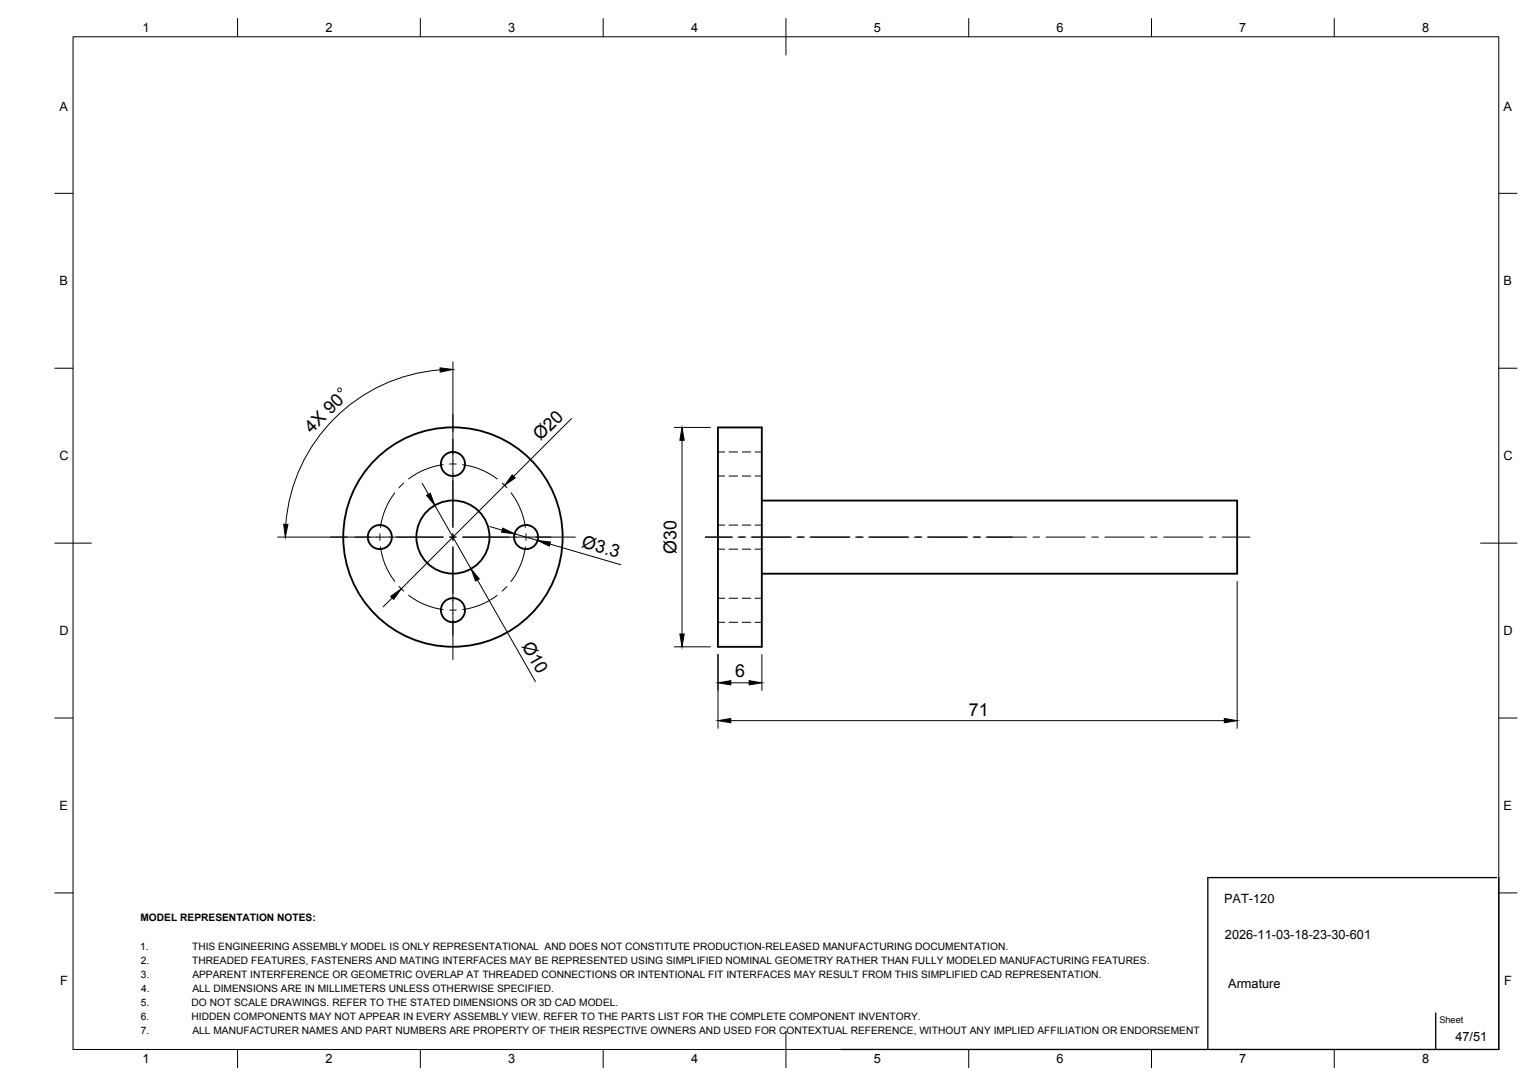
ISO-10303-21;
HEADER;
/* Generated by software containing ST-Developer
 * from STEP Tools, Inc. (www.steptools.com) 
 */

FILE_DESCRIPTION(
/* description */ ('Vibration shaker table dummy'),
/* implementation_level */ '2;1');

FILE_NAME(
/* name */ 'Armature.step',
/* time_stamp */ '2026-10-27T10:55:14-07:00',
/* author */ (''),
/* organization */ (''),
/* preprocessor_version */ 'ST-DEVELOPER v20.2',
/* originating_system */ 'Autodesk Translation Framework v15.17.0.0',
/* authorisation */ '');

FILE_SCHEMA (('AUTOMOTIVE_DESIGN { 1 0 10303 214 3 1 1 }'));
ENDSEC;

DATA;
#10=MECHANICAL_DESIGN_GEOMETRIC_PRESENTATION_REPRESENTATION('',(#728),#22394);
#636=SHAPE_REPRESENTATION_RELATIONSHIP('SRR','None',#22683,#682);
#682=ADVANCED_BREP_SHAPE_REPRESENTATION('',(#772),#22389);
#728=STYLED_ITEM('',(#22947),#772);
#772=MANIFOLD_SOLID_BREP('Body1',#9248);
#1039=FACE_BOUND('',#2555,.T.);
#1040=FACE_BOUND('',#2556,.T.);
#1041=FACE_BOUND('',#2557,.T.);
#1042=FACE_BOUND('',#2558,.T.);
#1043=FACE_BOUND('',#2559,.T.);
#1044=FACE_BOUND('',#2563,.T.);
#1045=FACE_BOUND('',#2564,.T.);
#1046=FACE_BOUND('',#2565,.T.);
#1047=FACE_BOUND('',#2566,.T.);
#1310=PLANE('',#10726);
#1311=PLANE('',#10733);
#1312=PLANE('',#10734);
#1788=FACE_OUTER_BOUND('',#2550,.T.);
#1789=FACE_OUTER_BOUND('',#2551,.T.);
#1790=FACE_OUTER_BOUND('',#2552,.T.);
#1791=FACE_OUTER_BOUND('',#2553,.T.);
#1792=FACE_OUTER_BOUND('',#2554,.T.);
#1793=FACE_OUTER_BOUND('',#2560,.T.);
#1794=FACE_OUTER_BOUND('',#2561,.T.);
#1795=FACE_OUTER_BOUND('',#2562,.T.);
#1796=FACE_OUTER_BOUND('',#2567,.T.);
#2550=EDGE_LOOP('',(#8310,#8311,#8312,#8313));
#2551=EDGE_LOOP('',(#8314,#8315,#8316,#8317));
#2552=EDGE_LOOP('',(#8318,#8319,#8320,#8321));
#2553=EDGE_LOOP('',(#8322,#8323,#8324,#8325));
#2554=EDGE_LOOP('',(#8326));
#2555=EDGE_LOOP('',(#8327));
#2556=EDGE_LOOP('',(#8328));
#2557=EDGE_LOOP('',(#8329));
#2558=EDGE_LOOP('',(#8330));
#2559=EDGE_LOOP('',(#8331));
#2560=EDGE_LOOP('',(#8332,#8333,#8334,#8335));
#2561=EDGE_LOOP('',(#8336,#8337,#8338,#8339));
#2562=EDGE_LOOP('',(#8340));
#2563=EDGE_LOOP('',(#8341));
#2564=EDGE_LOOP('',(#8342));
#2565=EDGE_LOOP('',(#8343));
#2566=EDGE_LOOP('',(#8344));
#2567=EDGE_LOOP('',(#8345));
#3185=LINE('',#21941,#3804);
#3186=LINE('',#21947,#3805);
#3187=LINE('',#21953,#3806);
#3188=LINE('',#21959,#3807);
#3189=LINE('',#21969,#3808);
#3190=LINE('',#21972,#3809);
#3804=VECTOR('',#13425,0.165);
#3805=VECTOR('',#13432,0.165);
#3806=VECTOR('',#13439,0.165);
#3807=VECTOR('',#13446,0.165);
#3808=VECTOR('',#13459,1.5);
#3809=VECTOR('',#13462,0.5);
#4325=CIRCLE('',#10715,0.165);
#4326=CIRCLE('',#10716,0.165);
#4327=CIRCLE('',#10718,0.165);
#4328=CIRCLE('',#10719,0.165);
#4329=CIRCLE('',#10721,0.165);
#4330=CIRCLE('',#10722,0.165);
#4331=CIRCLE('',#10724,0.165);
#4332=CIRCLE('',#10725,0.165);
#4333=CIRCLE('',#10727,1.5);
#4334=CIRCLE('',#10728,0.5);
#4335=CIRCLE('',#10730,1.5);
#4336=CIRCLE('',#10732,0.5);
#5052=VERTEX_POINT('',#21938);
#5053=VERTEX_POINT('',#21940);
#5054=VERTEX_POINT('',#21944);
#5055=VERTEX_POINT('',#21946);
#5056=VERTEX_POINT('',#21950);
#5057=VERTEX_POINT('',#21952);
#5058=VERTEX_POINT('',#21956);
#5059=VERTEX_POINT('',#21958);
#5060=VERTEX_POINT('',#21962);
#5061=VERTEX_POINT('',#21964);
#5062=VERTEX_POINT('',#21967);
#5063=VERTEX_POINT('',#21971);
#6148=EDGE_CURVE('',#5052,#5052,#4325,.T.);
#6149=EDGE_CURVE('',#5052,#5053,#3185,.T.);
#6150=EDGE_CURVE('',#5053,#5053,#4326,.T.);
#6151=EDGE_CURVE('',#5054,#5054,#4327,.T.);
#6152=EDGE_CURVE('',#5054,#5055,#3186,.T.);
#6153=EDGE_CURVE('',#5055,#5055,#4328,.T.);
#6154=EDGE_CURVE('',#5056,#5056,#4329,.T.);
#6155=EDGE_CURVE('',#5056,#5057,#3187,.T.);
#6156=EDGE_CURVE('',#5057,#5057,#4330,.T.);
#6157=EDGE_CURVE('',#5058,#5058,#4331,.T.);
#6158=EDGE_CURVE('',#5058,#5059,#3188,.T.);
#6159=EDGE_CURVE('',#5059,#5059,#4332,.T.);
#6160=EDGE_CURVE('',#5060,#5060,#4333,.T.);
#6161=EDGE_CURVE('',#5061,#5061,#4334,.T.);
#6162=EDGE_CURVE('',#5062,#5062,#4335,.T.);
#6163=EDGE_CURVE('',#5062,#5060,#3189,.T.);
#6164=EDGE_CURVE('',#5061,#5063,#3190,.T.);
#6165=EDGE_CURVE('',#5063,#5063,#4336,.T.);
#8310=ORIENTED_EDGE('',*,*,#6148,.F.);
#8311=ORIENTED_EDGE('',*,*,#6149,.T.);
#8312=ORIENTED_EDGE('',*,*,#6150,.F.);
#8313=ORIENTED_EDGE('',*,*,#6149,.F.);
#8314=ORIENTED_EDGE('',*,*,#6151,.F.);
#8315=ORIENTED_EDGE('',*,*,#6152,.T.);
#8316=ORIENTED_EDGE('',*,*,#6153,.F.);
#8317=ORIENTED_EDGE('',*,*,#6152,.F.);
#8318=ORIENTED_EDGE('',*,*,#6154,.F.);
#8319=ORIENTED_EDGE('',*,*,#6155,.T.);
#8320=ORIENTED_EDGE('',*,*,#6156,.F.);
#8321=ORIENTED_EDGE('',*,*,#6155,.F.);
#8322=ORIENTED_EDGE('',*,*,#6157,.F.);
#8323=ORIENTED_EDGE('',*,*,#6158,.T.);
#8324=ORIENTED_EDGE('',*,*,#6159,.F.);
#8325=ORIENTED_EDGE('',*,*,#6158,.F.);
#8326=ORIENTED_EDGE('',*,*,#6160,.F.);
#8327=ORIENTED_EDGE('',*,*,#6161,.F.);
#8328=ORIENTED_EDGE('',*,*,#6157,.T.);
#8329=ORIENTED_EDGE('',*,*,#6154,.T.);
#8330=ORIENTED_EDGE('',*,*,#6151,.T.);
#8331=ORIENTED_EDGE('',*,*,#6148,.T.);
#8332=ORIENTED_EDGE('',*,*,#6162,.F.);
#8333=ORIENTED_EDGE('',*,*,#6163,.T.);
#8334=ORIENTED_EDGE('',*,*,#6160,.T.);
#8335=ORIENTED_EDGE('',*,*,#6163,.F.);
#8336=ORIENTED_EDGE('',*,*,#6161,.T.);
#8337=ORIENTED_EDGE('',*,*,#6164,.T.);
#8338=ORIENTED_EDGE('',*,*,#6165,.T.);
#8339=ORIENTED_EDGE('',*,*,#6164,.F.);
#8340=ORIENTED_EDGE('',*,*,#6162,.T.);
#8341=ORIENTED_EDGE('',*,*,#6150,.T.);
#8342=ORIENTED_EDGE('',*,*,#6153,.T.);
#8343=ORIENTED_EDGE('',*,*,#6156,.T.);
#8344=ORIENTED_EDGE('',*,*,#6159,.T.);
#8345=ORIENTED_EDGE('',*,*,#6165,.F.);
#8690=CYLINDRICAL_SURFACE('',#10714,0.165);
#8691=CYLINDRICAL_SURFACE('',#10717,0.165);
#8692=CYLINDRICAL_SURFACE('',#10720,0.165);
#8693=CYLINDRICAL_SURFACE('',#10723,0.165);
#8694=CYLINDRICAL_SURFACE('',#10729,1.5);
#8695=CYLINDRICAL_SURFACE('',#10731,0.5);
#9153=ADVANCED_FACE('',(#1788),#8690,.F.);
#9154=ADVANCED_FACE('',(#1789),#8691,.F.);
#9155=ADVANCED_FACE('',(#1790),#8692,.F.);
#9156=ADVANCED_FACE('',(#1791),#8693,.F.);
#9157=ADVANCED_FACE('',(#1792,#1039,#1040,#1041,#1042,#1043),#1310,.F.);
#9158=ADVANCED_FACE('',(#1793),#8694,.T.);
#9159=ADVANCED_FACE('',(#1794),#8695,.T.);
#9160=ADVANCED_FACE('',(#1795,#1044,#1045,#1046,#1047),#1311,.T.);
#9161=ADVANCED_FACE('',(#1796),#1312,.F.);
#9248=CLOSED_SHELL('',(#9153,#9154,#9155,#9156,#9157,#9158,#9159,#9160,
#9161));
#10713=AXIS2_PLACEMENT_3D('',#21936,#13419,#13420);
#10714=AXIS2_PLACEMENT_3D('',#21937,#13421,#13422);
#10715=AXIS2_PLACEMENT_3D('',#21939,#13423,#13424);
#10716=AXIS2_PLACEMENT_3D('',#21942,#13426,#13427);
#10717=AXIS2_PLACEMENT_3D('',#21943,#13428,#13429);
#10718=AXIS2_PLACEMENT_3D('',#21945,#13430,#13431);
#10719=AXIS2_PLACEMENT_3D('',#21948,#13433,#13434);
#10720=AXIS2_PLACEMENT_3D('',#21949,#13435,#13436);
#10721=AXIS2_PLACEMENT_3D('',#21951,#13437,#13438);
#10722=AXIS2_PLACEMENT_3D('',#21954,#13440,#13441);
#10723=AXIS2_PLACEMENT_3D('',#21955,#13442,#13443);
#10724=AXIS2_PLACEMENT_3D('',#21957,#13444,#13445);
#10725=AXIS2_PLACEMENT_3D('',#21960,#13447,#13448);
#10726=AXIS2_PLACEMENT_3D('',#21961,#13449,#13450);
#10727=AXIS2_PLACEMENT_3D('',#21963,#13451,#13452);
#10728=AXIS2_PLACEMENT_3D('',#21965,#13453,#13454);
#10729=AXIS2_PLACEMENT_3D('',#21966,#13455,#13456);
#10730=AXIS2_PLACEMENT_3D('',#21968,#13457,#13458);
#10731=AXIS2_PLACEMENT_3D('',#21970,#13460,#13461);
#10732=AXIS2_PLACEMENT_3D('',#21973,#13463,#13464);
#10733=AXIS2_PLACEMENT_3D('',#21974,#13465,#13466);
#10734=AXIS2_PLACEMENT_3D('',#21975,#13467,#13468);
#13419=DIRECTION('axis',(0.,0.,1.));
#13420=DIRECTION('refdir',(1.,0.,0.));
#13421=DIRECTION('center_axis',(0.,0.,1.));
#13422=DIRECTION('ref_axis',(1.,0.,0.));
#13423=DIRECTION('center_axis',(0.,0.,1.));
#13424=DIRECTION('ref_axis',(1.,0.,0.));
#13425=DIRECTION('',(0.,0.,1.));
#13426=DIRECTION('center_axis',(0.,0.,-1.));
#13427=DIRECTION('ref_axis',(1.,0.,0.));
#13428=DIRECTION('center_axis',(0.,0.,1.));
#13429=DIRECTION('ref_axis',(1.,0.,0.));
#13430=DIRECTION('center_axis',(0.,0.,1.));
#13431=DIRECTION('ref_axis',(1.,0.,0.));
#13432=DIRECTION('',(0.,0.,1.));
#13433=DIRECTION('center_axis',(0.,0.,-1.));
#13434=DIRECTION('ref_axis',(1.,0.,0.));
#13435=DIRECTION('center_axis',(0.,0.,1.));
#13436=DIRECTION('ref_axis',(1.,0.,0.));
#13437=DIRECTION('center_axis',(0.,0.,1.));
#13438=DIRECTION('ref_axis',(1.,0.,0.));
#13439=DIRECTION('',(0.,0.,1.));
#13440=DIRECTION('center_axis',(0.,0.,-1.));
#13441=DIRECTION('ref_axis',(1.,0.,0.));
#13442=DIRECTION('center_axis',(0.,0.,1.));
#13443=DIRECTION('ref_axis',(1.,0.,0.));
#13444=DIRECTION('center_axis',(0.,0.,1.));
#13445=DIRECTION('ref_axis',(1.,0.,0.));
#13446=DIRECTION('',(0.,0.,1.));
#13447=DIRECTION('center_axis',(0.,0.,-1.));
#13448=DIRECTION('ref_axis',(1.,0.,0.));
#13449=DIRECTION('center_axis',(0.,0.,1.));
#13450=DIRECTION('ref_axis',(1.,0.,0.));
#13451=DIRECTION('center_axis',(0.,0.,1.));
#13452=DIRECTION('ref_axis',(1.,0.,0.));
#13453=DIRECTION('center_axis',(0.,0.,-1.));
#13454=DIRECTION('ref_axis',(1.,0.,0.));
#13455=DIRECTION('center_axis',(0.,0.,1.));
#13456=DIRECTION('ref_axis',(1.,0.,0.));
#13457=DIRECTION('center_axis',(0.,0.,1.));
#13458=DIRECTION('ref_axis',(1.,0.,0.));
#13459=DIRECTION('',(0.,0.,-1.));
#13460=DIRECTION('center_axis',(0.,0.,1.));
#13461=DIRECTION('ref_axis',(1.,0.,0.));
#13462=DIRECTION('',(0.,0.,-1.));
#13463=DIRECTION('center_axis',(0.,0.,1.));
#13464=DIRECTION('ref_axis',(1.,0.,0.));
#13465=DIRECTION('center_axis',(0.,0.,1.));
#13466=DIRECTION('ref_axis',(1.,0.,0.));
#13467=DIRECTION('center_axis',(0.,0.,1.));
#13468=DIRECTION('ref_axis',(1.,0.,0.));
#21936=CARTESIAN_POINT('',(0.,0.,0.));
#21937=CARTESIAN_POINT('Origin',(0.,-1.,14.4));
#21938=CARTESIAN_POINT('',(-0.165,-1.,14.5));
#21939=CARTESIAN_POINT('Origin',(0.,-1.,14.5));
#21940=CARTESIAN_POINT('',(-0.165,-1.,15.1));
#21941=CARTESIAN_POINT('',(-0.165,-1.,14.4));
#21942=CARTESIAN_POINT('Origin',(0.,-1.,15.1));
#21943=CARTESIAN_POINT('Origin',(1.,0.,14.4));
#21944=CARTESIAN_POINT('',(0.835,-2.02066721859313E-17,14.5));
#21945=CARTESIAN_POINT('Origin',(1.,0.,14.5));
#21946=CARTESIAN_POINT('',(0.835,2.02066721859313E-17,15.1));
#21947=CARTESIAN_POINT('',(0.835,-2.02066721859313E-17,14.4));
#21948=CARTESIAN_POINT('Origin',(1.,0.,15.1));
#21949=CARTESIAN_POINT('Origin',(-1.,0.,14.4));
#21950=CARTESIAN_POINT('',(-1.165,-2.02066721859313E-17,14.5));
#21951=CARTESIAN_POINT('Origin',(-1.,0.,14.5));
#21952=CARTESIAN_POINT('',(-1.165,2.02066721859313E-17,15.1));
#21953=CARTESIAN_POINT('',(-1.165,-2.02066721859313E-17,14.4));
#21954=CARTESIAN_POINT('Origin',(-1.,0.,15.1));
#21955=CARTESIAN_POINT('Origin',(0.,1.,14.4));
#21956=CARTESIAN_POINT('',(-0.165,1.,14.5));
#21957=CARTESIAN_POINT('Origin',(0.,1.,14.5));
#21958=CARTESIAN_POINT('',(-0.165,1.,15.1));
#21959=CARTESIAN_POINT('',(-0.165,1.,14.4));
#21960=CARTESIAN_POINT('Origin',(0.,1.,15.1));
#21961=CARTESIAN_POINT('Origin',(0.,0.,14.5));
#21962=CARTESIAN_POINT('',(-1.5,-1.83697019872103E-16,14.5));
#21963=CARTESIAN_POINT('Origin',(0.,0.,14.5));
#21964=CARTESIAN_POINT('',(-0.5,6.12323399573677E-17,14.5));
#21965=CARTESIAN_POINT('Origin',(0.,0.,14.5));
#21966=CARTESIAN_POINT('Origin',(0.,0.,14.5));
#21967=CARTESIAN_POINT('',(-1.5,-1.83697019872103E-16,15.1));
#21968=CARTESIAN_POINT('Origin',(0.,0.,15.1));
#21969=CARTESIAN_POINT('',(-1.5,-1.83697019872103E-16,14.5));
#21970=CARTESIAN_POINT('Origin',(0.,0.,8.));
#21971=CARTESIAN_POINT('',(-0.5,-6.12323399573677E-17,8.));
#21972=CARTESIAN_POINT('',(-0.5,-6.12323399573677E-17,8.));
#21973=CARTESIAN_POINT('Origin',(0.,0.,8.));
#21974=CARTESIAN_POINT('Origin',(0.,0.,15.1));
#21975=CARTESIAN_POINT('Origin',(0.,0.,8.));
#22338=UNCERTAINTY_MEASURE_WITH_UNIT(LENGTH_MEASURE(0.001),#22395,
'DISTANCE_ACCURACY_VALUE',
'Maximum model space distance between geometric entities at asserted c
onnectivities');
#22343=UNCERTAINTY_MEASURE_WITH_UNIT(LENGTH_MEASURE(0.001),#22395,
'DISTANCE_ACCURACY_VALUE',
'Maximum model space distance between geometric entities at asserted c
onnectivities');
#22389=(
GEOMETRIC_REPRESENTATION_CONTEXT(3)
GLOBAL_UNCERTAINTY_ASSIGNED_CONTEXT((#22338))
GLOBAL_UNIT_ASSIGNED_CONTEXT((#22395,#22397,#22398))
REPRESENTATION_CONTEXT('','3D')
);
#22394=(
GEOMETRIC_REPRESENTATION_CONTEXT(3)
GLOBAL_UNCERTAINTY_ASSIGNED_CONTEXT((#22343))
GLOBAL_UNIT_ASSIGNED_CONTEXT((#22395,#22397,#22398))
REPRESENTATION_CONTEXT('','3D')
);
#22395=(
LENGTH_UNIT()
NAMED_UNIT(*)
SI_UNIT(.CENTI.,.METRE.)
);
#22397=(
NAMED_UNIT(*)
PLANE_ANGLE_UNIT()
SI_UNIT($,.RADIAN.)
);
#22398=(
NAMED_UNIT(*)
SI_UNIT($,.STERADIAN.)
SOLID_ANGLE_UNIT()
);
#22444=SHAPE_DEFINITION_REPRESENTATION(#22494,#22683);
#22494=PRODUCT_DEFINITION_SHAPE('',$,#22734);
#22683=SHAPE_REPRESENTATION('',(#10713),#22389);
#22688=PRODUCT_DEFINITION_CONTEXT('part definition',#22840,'design');
#22734=PRODUCT_DEFINITION('Armature','Armature',#22784,#22688);
#22784=PRODUCT_DEFINITION_FORMATION('',$,#22887);
#22840=APPLICATION_CONTEXT(
'Core Data for Automotive Mechanical Design Process');
#22841=PRODUCT_CONTEXT('part definition',#22840,'mechanical');
#22887=PRODUCT('Armature','Armature','Armature',(#22841));
#22941=COLOUR_RGB('Light Blue',0.38,0.62,0.78);
#22942=FILL_AREA_STYLE_COLOUR('',#22941);
#22943=FILL_AREA_STYLE('',(#22942));
#22944=SURFACE_STYLE_FILL_AREA(#22943);
#22945=SURFACE_SIDE_STYLE('',(#22944));
#22946=SURFACE_STYLE_USAGE(.BOTH.,#22945);
#22947=PRESENTATION_STYLE_ASSIGNMENT((#22946));
ENDSEC;
END-ISO-10303-21;
